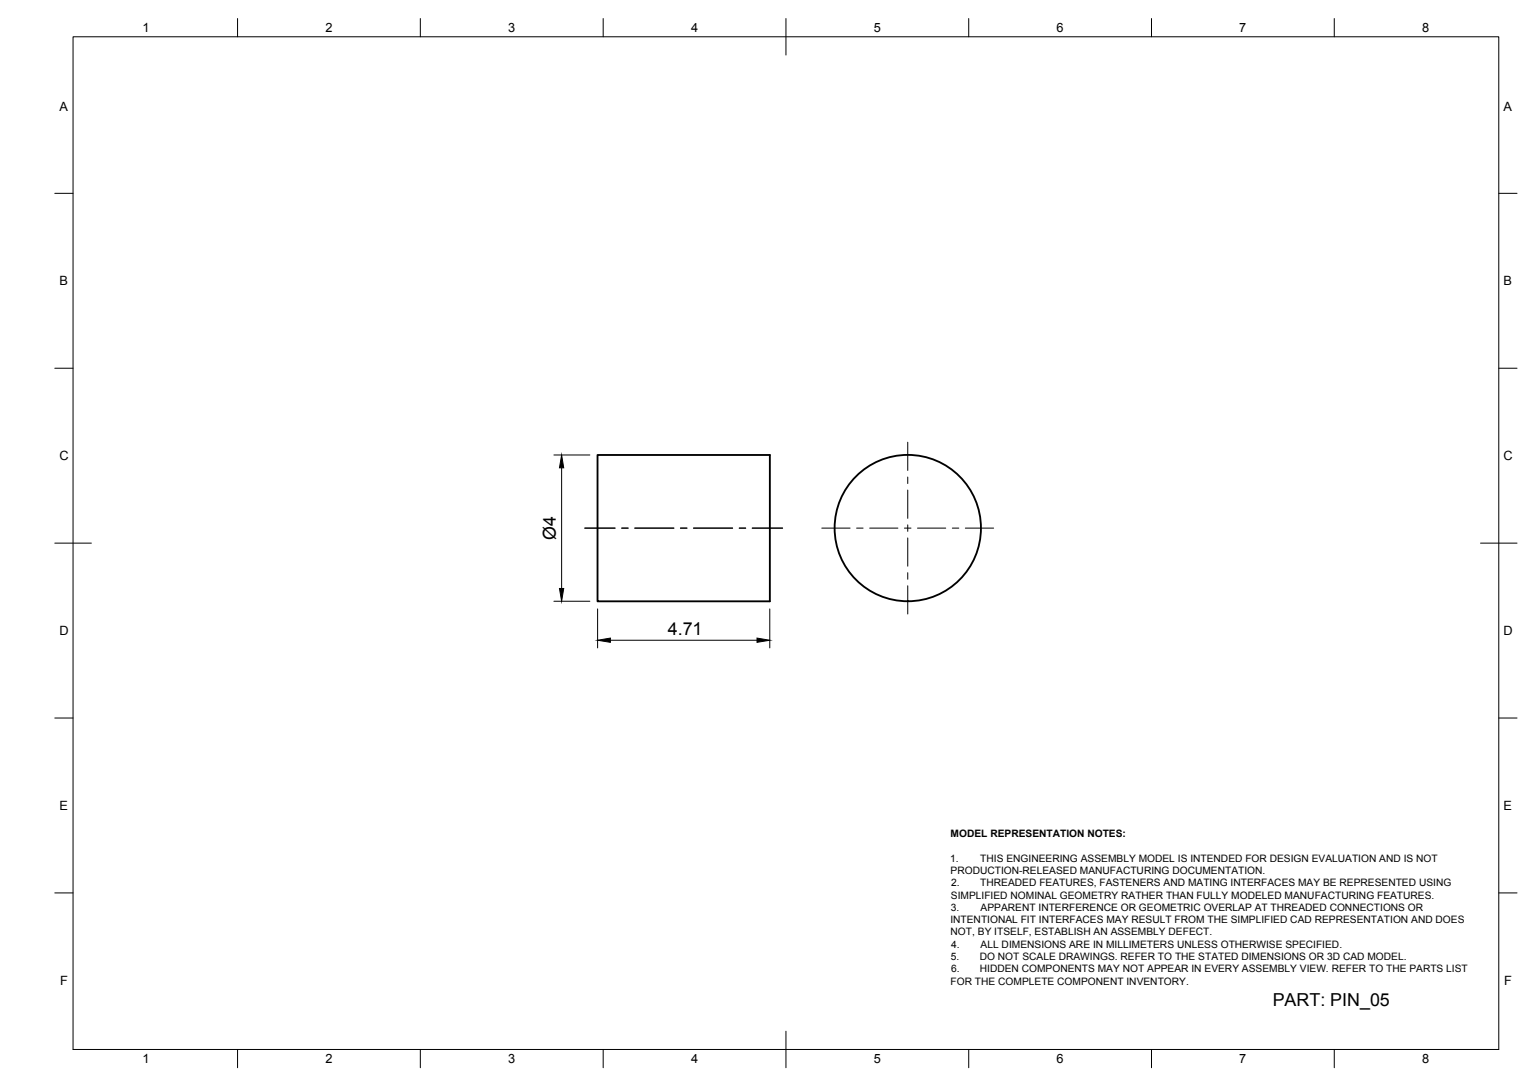
ISO-10303-21;
HEADER;
/* Generated by software containing ST-Developer
 * from STEP Tools, Inc. (www.steptools.com) 
 */

FILE_DESCRIPTION(
/* description */ (''),
/* implementation_level */ '2;1');

FILE_NAME(
/* name */ 'Pin_05.step',
/* time_stamp */ '2026-10-05T13:12:53-07:00',
/* author */ (''),
/* organization */ (''),
/* preprocessor_version */ 'ST-DEVELOPER v20.2',
/* originating_system */ 'Autodesk Translation Framework v15.15.0.0',
/* authorisation */ '');

FILE_SCHEMA (('AUTOMOTIVE_DESIGN { 1 0 10303 214 3 1 1 }'));
ENDSEC;

DATA;
#10=MECHANICAL_DESIGN_GEOMETRIC_PRESENTATION_REPRESENTATION('',(#64),#5912);
#48=SHAPE_REPRESENTATION_RELATIONSHIP('SRR','None',#5949,#56);
#56=ADVANCED_BREP_SHAPE_REPRESENTATION('',(#72),#5909);
#64=STYLED_ITEM('',(#5994),#72);
#72=MANIFOLD_SOLID_BREP('Body1',#3475);
#165=CYLINDRICAL_SURFACE('',#3861,2.);
#341=FACE_OUTER_BOUND('',#544,.T.);
#342=FACE_OUTER_BOUND('',#545,.T.);
#343=FACE_OUTER_BOUND('',#546,.T.);
#544=EDGE_LOOP('',(#3142,#3143,#3144,#3145));
#545=EDGE_LOOP('',(#3146));
#546=EDGE_LOOP('',(#3147));
#649=CIRCLE('',#3862,2.);
#650=CIRCLE('',#3863,2.);
#1017=LINE('',#5863,#1382);
#1382=VECTOR('',#4840,2.);
#1699=VERTEX_POINT('',#5860);
#1700=VERTEX_POINT('',#5862);
#2181=EDGE_CURVE('',#1699,#1699,#649,.T.);
#2182=EDGE_CURVE('',#1699,#1700,#1017,.T.);
#2183=EDGE_CURVE('',#1700,#1700,#650,.T.);
#3142=ORIENTED_EDGE('',*,*,#2181,.F.);
#3143=ORIENTED_EDGE('',*,*,#2182,.T.);
#3144=ORIENTED_EDGE('',*,*,#2183,.F.);
#3145=ORIENTED_EDGE('',*,*,#2182,.F.);
#3146=ORIENTED_EDGE('',*,*,#2183,.T.);
#3147=ORIENTED_EDGE('',*,*,#2181,.T.);
#3282=PLANE('',#3864);
#3283=PLANE('',#3865);
#3461=ADVANCED_FACE('',(#341),#165,.T.);
#3462=ADVANCED_FACE('',(#342),#3282,.T.);
#3463=ADVANCED_FACE('',(#343),#3283,.F.);
#3475=CLOSED_SHELL('',(#3461,#3462,#3463));
#3860=AXIS2_PLACEMENT_3D('',#5858,#4834,#4835);
#3861=AXIS2_PLACEMENT_3D('',#5859,#4836,#4837);
#3862=AXIS2_PLACEMENT_3D('',#5861,#4838,#4839);
#3863=AXIS2_PLACEMENT_3D('',#5864,#4841,#4842);
#3864=AXIS2_PLACEMENT_3D('',#5865,#4843,#4844);
#3865=AXIS2_PLACEMENT_3D('',#5866,#4845,#4846);
#4834=DIRECTION('axis',(0.,0.,1.));
#4835=DIRECTION('refdir',(1.,0.,0.));
#4836=DIRECTION('center_axis',(0.,0.0208291764396898,-0.999783049170591));
#4837=DIRECTION('ref_axis',(1.,0.,0.));
#4838=DIRECTION('center_axis',(0.,0.0208291764396898,-0.999783049170591));
#4839=DIRECTION('ref_axis',(1.,0.,0.));
#4840=DIRECTION('',(0.,-0.0208291764396898,0.999783049170591));
#4841=DIRECTION('center_axis',(0.,-0.0208291764396898,0.999783049170591));
#4842=DIRECTION('ref_axis',(1.,0.,0.));
#4843=DIRECTION('center_axis',(0.,-0.0208291764396898,0.999783049170591));
#4844=DIRECTION('ref_axis',(1.,0.,0.));
#4845=DIRECTION('center_axis',(0.,-0.0208291764396898,0.999783049170591));
#4846=DIRECTION('ref_axis',(1.,0.,0.));
#5858=CARTESIAN_POINT('',(0.,0.,0.));
#5859=CARTESIAN_POINT('Origin',(55.4902124404907,-12.0000001341105,105.854167938232));
#5860=CARTESIAN_POINT('',(53.4902124404907,-11.9018738839031,101.14418999359));
#5861=CARTESIAN_POINT('Origin',(55.4902124404907,-11.9018738839031,101.14418999359));
#5862=CARTESIAN_POINT('',(53.4902124404907,-12.0000001341105,105.854167938232));
#5863=CARTESIAN_POINT('',(53.4902124404907,-12.0000001341105,105.854167938232));
#5864=CARTESIAN_POINT('Origin',(55.4902124404907,-12.0000001341105,105.854167938232));
#5865=CARTESIAN_POINT('Origin',(55.4902124404907,-12.0000001341105,105.854167938232));
#5866=CARTESIAN_POINT('Origin',(55.4902124404907,-11.9018738839031,101.14418999359));
#5899=UNCERTAINTY_MEASURE_WITH_UNIT(LENGTH_MEASURE(0.01),#5913,
'DISTANCE_ACCURACY_VALUE',
'Maximum model space distance between geometric entities at asserted c
onnectivities');
#5902=UNCERTAINTY_MEASURE_WITH_UNIT(LENGTH_MEASURE(0.01),#5913,
'DISTANCE_ACCURACY_VALUE',
'Maximum model space distance between geometric entities at asserted c
onnectivities');
#5909=(
GEOMETRIC_REPRESENTATION_CONTEXT(3)
GLOBAL_UNCERTAINTY_ASSIGNED_CONTEXT((#5899))
GLOBAL_UNIT_ASSIGNED_CONTEXT((#5913,#5915,#5916))
REPRESENTATION_CONTEXT('','3D')
);
#5912=(
GEOMETRIC_REPRESENTATION_CONTEXT(3)
GLOBAL_UNCERTAINTY_ASSIGNED_CONTEXT((#5902))
GLOBAL_UNIT_ASSIGNED_CONTEXT((#5913,#5915,#5916))
REPRESENTATION_CONTEXT('','3D')
);
#5913=(
LENGTH_UNIT()
NAMED_UNIT(*)
SI_UNIT(.MILLI.,.METRE.)
);
#5915=(
NAMED_UNIT(*)
PLANE_ANGLE_UNIT()
SI_UNIT($,.RADIAN.)
);
#5916=(
NAMED_UNIT(*)
SI_UNIT($,.STERADIAN.)
SOLID_ANGLE_UNIT()
);
#5923=SHAPE_DEFINITION_REPRESENTATION(#5932,#5949);
#5932=PRODUCT_DEFINITION_SHAPE('',$,#5959);
#5949=SHAPE_REPRESENTATION('',(#3860),#5909);
#5952=PRODUCT_DEFINITION_CONTEXT('part definition',#5981,'design');
#5959=PRODUCT_DEFINITION('Pin_05','Pin_05',#5968,#5952);
#5968=PRODUCT_DEFINITION_FORMATION('',$,#5989);
#5981=APPLICATION_CONTEXT(
'Core Data for Automotive Mechanical Design Process');
#5982=PRODUCT_CONTEXT('part definition',#5981,'mechanical');
#5989=PRODUCT('Pin_05','Pin_05',$,(#5982));
#5994=PRESENTATION_STYLE_ASSIGNMENT((#5997));
#5997=SURFACE_STYLE_USAGE(.BOTH.,#6000);
#6000=SURFACE_SIDE_STYLE('',(#6003));
#6003=SURFACE_STYLE_FILL_AREA(#6006);
#6006=FILL_AREA_STYLE('Opaque(160,160,160)',(#6009));
#6009=FILL_AREA_STYLE_COLOUR('Opaque(160,160,160)',#6012);
#6012=COLOUR_RGB('Opaque(160,160,160)', 0.31764706, 0.68627451, 0.89019608);
ENDSEC;
END-ISO-10303-21;
